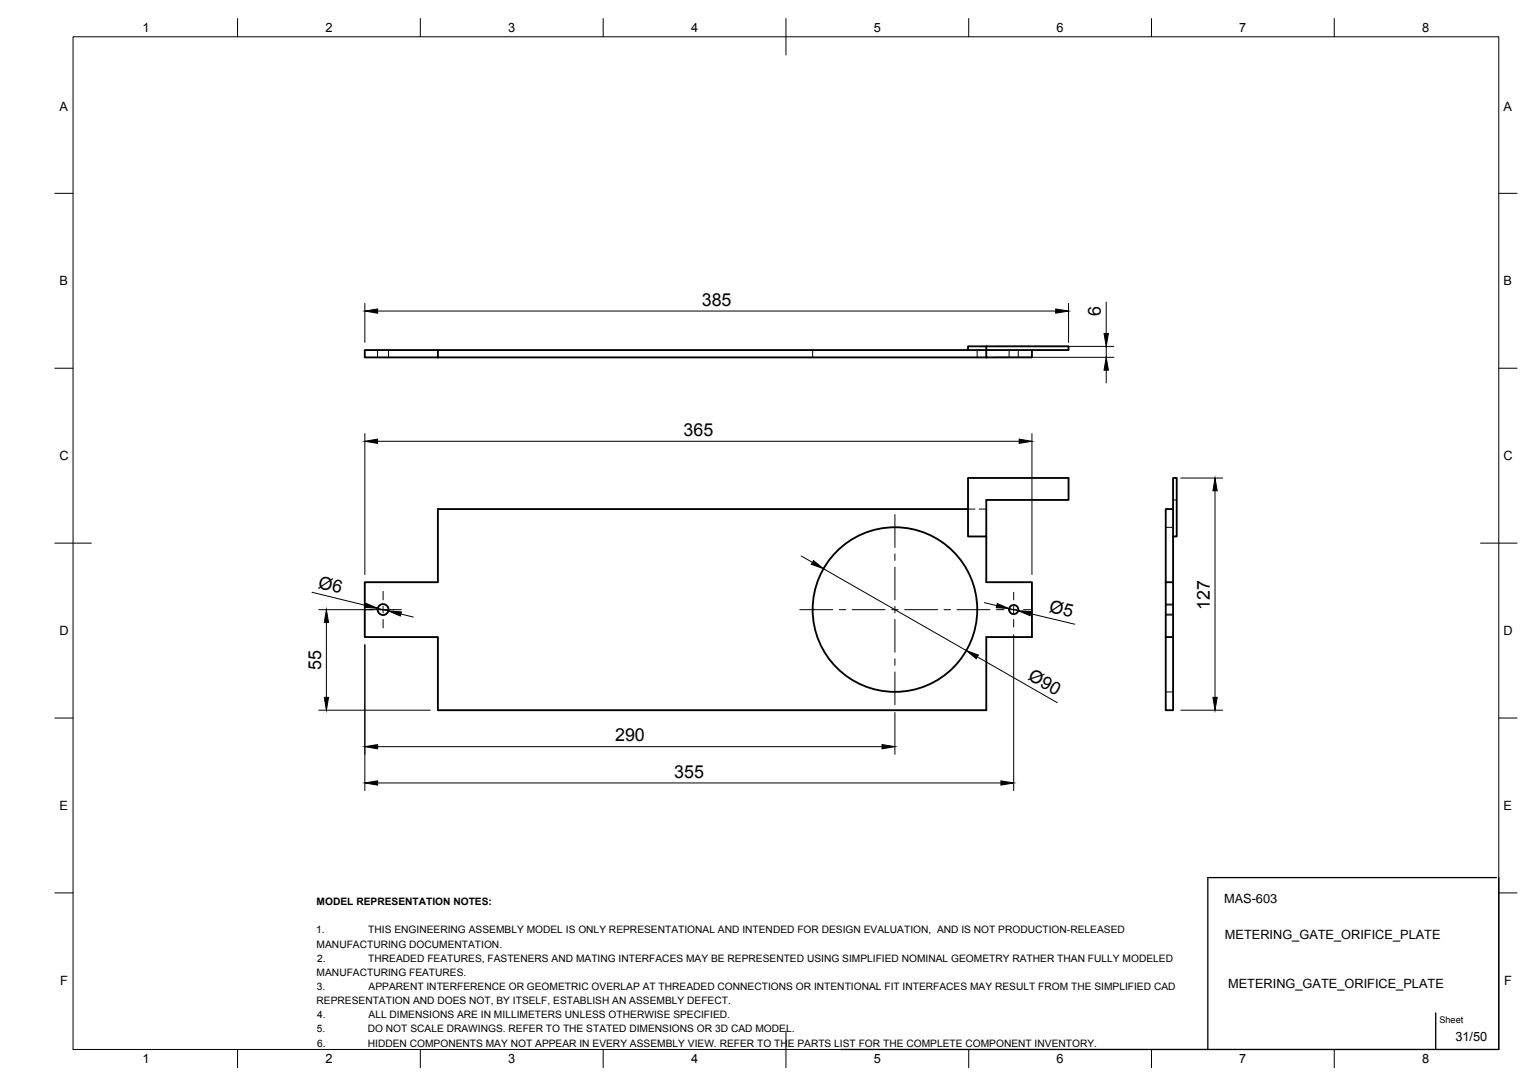
ISO-10303-21;
HEADER;
FILE_DESCRIPTION((''),'2;1');
FILE_NAME('METERING_GATE_ORIFICE_PLATE.step','2026-10-01T22:06:14-07:00',(''),(''),'','','');
FILE_SCHEMA (('AUTOMOTIVE_DESIGN { 1 0 10303 214 3 1 1 }'));
ENDSEC;
DATA;
#10=MECHANICAL_DESIGN_GEOMETRIC_PRESENTATION_REPRESENTATION('',(#1003),#50440);
#911=SHAPE_REPRESENTATION_RELATIONSHIP('SRR','None',#50644,#956) ;
#956=ADVANCED_BREP_SHAPE_REPRESENTATION('',(#1058),#50413) ;
#1003=STYLED_ITEM('',(#50889),#1058) ;
#1058=MANIFOLD_SOLID_BREP('METERING_GATE_ORIFICE_PLATE',#28670) ;
#1332=FACE_BOUND('',#5081,.T.) ;
#1333=FACE_BOUND('',#5082,.T.) ;
#1334=FACE_BOUND('',#5083,.T.) ;
#1335=FACE_BOUND('',#5085,.T.) ;
#1336=FACE_BOUND('',#5086,.T.) ;
#1337=FACE_BOUND('',#5087,.T.) ;
#2131=PLANE('',#30735) ;
#2132=PLANE('',#30736) ;
#2133=PLANE('',#30737) ;
#2134=PLANE('',#30738) ;
#2135=PLANE('',#30739) ;
#2136=PLANE('',#30740) ;
#2137=PLANE('',#30741) ;
#2138=PLANE('',#30745) ;
#2139=PLANE('',#30746) ;
#2140=PLANE('',#30747) ;
#2141=PLANE('',#30748) ;
#2142=PLANE('',#30749) ;
#2143=PLANE('',#30753) ;
#2144=PLANE('',#30754) ;
#2145=PLANE('',#30755) ;
#2146=PLANE('',#30756) ;
#2147=PLANE('',#30757) ;
#2148=PLANE('',#30761) ;
#2149=PLANE('',#30762) ;
#2150=PLANE('',#30763) ;
#2151=PLANE('',#30764) ;
#3286=FACE_OUTER_BOUND('',#5060,.T.) ;
#3287=FACE_OUTER_BOUND('',#5061,.T.) ;
#3288=FACE_OUTER_BOUND('',#5062,.T.) ;
#3289=FACE_OUTER_BOUND('',#5063,.T.) ;
#3290=FACE_OUTER_BOUND('',#5064,.T.) ;
#3291=FACE_OUTER_BOUND('',#5065,.T.) ;
#3292=FACE_OUTER_BOUND('',#5066,.T.) ;
#3293=FACE_OUTER_BOUND('',#5067,.T.) ;
#3294=FACE_OUTER_BOUND('',#5068,.T.) ;
#3295=FACE_OUTER_BOUND('',#5069,.T.) ;
#3296=FACE_OUTER_BOUND('',#5070,.T.) ;
#3297=FACE_OUTER_BOUND('',#5071,.T.) ;
#3298=FACE_OUTER_BOUND('',#5072,.T.) ;
#3299=FACE_OUTER_BOUND('',#5073,.T.) ;
#3300=FACE_OUTER_BOUND('',#5074,.T.) ;
#3301=FACE_OUTER_BOUND('',#5075,.T.) ;
#3302=FACE_OUTER_BOUND('',#5076,.T.) ;
#3303=FACE_OUTER_BOUND('',#5077,.T.) ;
#3304=FACE_OUTER_BOUND('',#5078,.T.) ;
#3305=FACE_OUTER_BOUND('',#5079,.T.) ;
#3306=FACE_OUTER_BOUND('',#5080,.T.) ;
#3307=FACE_OUTER_BOUND('',#5084,.T.) ;
#3308=FACE_OUTER_BOUND('',#5088,.T.) ;
#3309=FACE_OUTER_BOUND('',#5089,.T.) ;
#5060=EDGE_LOOP('',(#23447,#23448,#23449,#23450)) ;
#5061=EDGE_LOOP('',(#23451,#23452,#23453,#23454)) ;
#5062=EDGE_LOOP('',(#23455,#23456,#23457,#23458,#23459,#23460)) ;
#5063=EDGE_LOOP('',(#23461,#23462,#23463,#23464,#23465)) ;
#5064=EDGE_LOOP('',(#23466,#23467,#23468,#23469,#23470,#23471)) ;
#5065=EDGE_LOOP('',(#23472,#23473,#23474,#23475)) ;
#5066=EDGE_LOOP('',(#23476,#23477,#23478,#23479)) ;
#5067=EDGE_LOOP('',(#23480,#23481,#23482,#23483)) ;
#5068=EDGE_LOOP('',(#23484,#23485,#23486,#23487)) ;
#5069=EDGE_LOOP('',(#23488,#23489,#23490,#23491)) ;
#5070=EDGE_LOOP('',(#23492,#23493,#23494,#23495)) ;
#5071=EDGE_LOOP('',(#23496,#23497,#23498,#23499)) ;
#5072=EDGE_LOOP('',(#23500,#23501,#23502,#23503,#23504,#23505,#23506,#23507)) ;
#5073=EDGE_LOOP('',(#23508,#23509,#23510,#23511)) ;
#5074=EDGE_LOOP('',(#23512,#23513,#23514,#23515)) ;
#5075=EDGE_LOOP('',(#23516,#23517,#23518,#23519)) ;
#5076=EDGE_LOOP('',(#23520,#23521,#23522,#23523)) ;
#5077=EDGE_LOOP('',(#23524,#23525,#23526,#23527)) ;
#5078=EDGE_LOOP('',(#23528,#23529,#23530,#23531)) ;
#5079=EDGE_LOOP('',(#23532,#23533,#23534,#23535)) ;
#5080=EDGE_LOOP('',(#23536,#23537,#23538,#23539,#23540,#23541,#23542,#23543,
#23544,#23545,#23546,#23547,#23548,#23549)) ;
#5081=EDGE_LOOP('',(#23550)) ;
#5082=EDGE_LOOP('',(#23551)) ;
#5083=EDGE_LOOP('',(#23552)) ;
#5084=EDGE_LOOP('',(#23553,#23554,#23555,#23556,#23557,#23558,#23559,#23560,
#23561,#23562,#23563,#23564)) ;
#5085=EDGE_LOOP('',(#23565)) ;
#5086=EDGE_LOOP('',(#23566)) ;
#5087=EDGE_LOOP('',(#23567)) ;
#5088=EDGE_LOOP('',(#23568,#23569,#23570,#23571)) ;
#5089=EDGE_LOOP('',(#23572,#23573,#23574,#23575,#23576)) ;
#7620=LINE('',#46428,#10092) ;
#7621=LINE('',#46430,#10093) ;
#7622=LINE('',#46432,#10094) ;
#7623=LINE('',#46433,#10095) ;
#7624=LINE('',#46436,#10096) ;
#7625=LINE('',#46438,#10097) ;
#7626=LINE('',#46439,#10098) ;
#7627=LINE('',#46443,#10099) ;
#7628=LINE('',#46445,#10100) ;
#7629=LINE('',#46446,#10101) ;
#7630=LINE('',#46447,#10102) ;
#7631=LINE('',#46451,#10103) ;
#7632=LINE('',#46452,#10104) ;
#7633=LINE('',#46454,#10105) ;
#7634=LINE('',#46455,#10106) ;
#7635=LINE('',#46458,#10107) ;
#7636=LINE('',#46459,#10108) ;
#7637=LINE('',#46460,#10109) ;
#7638=LINE('',#46463,#10110) ;
#7639=LINE('',#46464,#10111) ;
#7640=LINE('',#46470,#10112) ;
#7641=LINE('',#46475,#10113) ;
#7642=LINE('',#46477,#10114) ;
#7643=LINE('',#46479,#10115) ;
#7644=LINE('',#46480,#10116) ;
#7645=LINE('',#46484,#10117) ;
#7646=LINE('',#46486,#10118) ;
#7647=LINE('',#46488,#10119) ;
#7648=LINE('',#46489,#10120) ;
#7649=LINE('',#46491,#10121) ;
#7650=LINE('',#46492,#10122) ;
#7651=LINE('',#46495,#10123) ;
#7652=LINE('',#46497,#10124) ;
#7653=LINE('',#46498,#10125) ;
#7654=LINE('',#46501,#10126) ;
#7655=LINE('',#46502,#10127) ;
#7656=LINE('',#46503,#10128) ;
#7657=LINE('',#46508,#10129) ;
#7658=LINE('',#46513,#10130) ;
#7659=LINE('',#46515,#10131) ;
#7660=LINE('',#46517,#10132) ;
#7661=LINE('',#46518,#10133) ;
#7662=LINE('',#46522,#10134) ;
#7663=LINE('',#46523,#10135) ;
#7664=LINE('',#46524,#10136) ;
#7665=LINE('',#46528,#10137) ;
#7666=LINE('',#46529,#10138) ;
#7667=LINE('',#46530,#10139) ;
#7668=LINE('',#46533,#10140) ;
#7669=LINE('',#46535,#10141) ;
#7670=LINE('',#46536,#10142) ;
#7671=LINE('',#46539,#10143) ;
#7672=LINE('',#46541,#10144) ;
#7673=LINE('',#46542,#10145) ;
#7674=LINE('',#46547,#10146) ;
#7675=LINE('',#46550,#10147) ;
#7676=LINE('',#46551,#10148) ;
#7677=LINE('',#46553,#10149) ;
#7678=LINE('',#46554,#10150) ;
#10092=VECTOR('',#37317,1.) ;
#10093=VECTOR('',#37318,1.) ;
#10094=VECTOR('',#37319,1.) ;
#10095=VECTOR('',#37320,1.) ;
#10096=VECTOR('',#37323,1.) ;
#10097=VECTOR('',#37324,1.) ;
#10098=VECTOR('',#37325,1.) ;
#10099=VECTOR('',#37328,1.) ;
#10100=VECTOR('',#37329,1.) ;
#10101=VECTOR('',#37330,1.) ;
#10102=VECTOR('',#37331,1.) ;
#10103=VECTOR('',#37334,1.) ;
#10104=VECTOR('',#37335,1.) ;
#10105=VECTOR('',#37336,1.) ;
#10106=VECTOR('',#37337,1.) ;
#10107=VECTOR('',#37340,1.) ;
#10108=VECTOR('',#37341,1.) ;
#10109=VECTOR('',#37342,1.) ;
#10110=VECTOR('',#37345,1.) ;
#10111=VECTOR('',#37346,1.) ;
#10112=VECTOR('',#37353,0.25) ;
#10113=VECTOR('',#37358,1.) ;
#10114=VECTOR('',#37359,1.) ;
#10115=VECTOR('',#37360,1.) ;
#10116=VECTOR('',#37361,1.) ;
#10117=VECTOR('',#37364,1.) ;
#10118=VECTOR('',#37365,1.) ;
#10119=VECTOR('',#37366,1.) ;
#10120=VECTOR('',#37367,1.) ;
#10121=VECTOR('',#37370,1.) ;
#10122=VECTOR('',#37371,1.) ;
#10123=VECTOR('',#37374,1.) ;
#10124=VECTOR('',#37375,1.) ;
#10125=VECTOR('',#37376,1.) ;
#10126=VECTOR('',#37379,1.) ;
#10127=VECTOR('',#37380,1.) ;
#10128=VECTOR('',#37381,1.) ;
#10129=VECTOR('',#37386,0.3) ;
#10130=VECTOR('',#37391,1.) ;
#10131=VECTOR('',#37392,1.) ;
#10132=VECTOR('',#37393,1.) ;
#10133=VECTOR('',#37394,1.) ;
#10134=VECTOR('',#37397,1.) ;
#10135=VECTOR('',#37398,1.) ;
#10136=VECTOR('',#37399,1.) ;
#10137=VECTOR('',#37402,1.) ;
#10138=VECTOR('',#37403,1.) ;
#10139=VECTOR('',#37404,1.) ;
#10140=VECTOR('',#37407,1.) ;
#10141=VECTOR('',#37408,1.) ;
#10142=VECTOR('',#37409,1.) ;
#10143=VECTOR('',#37412,1.) ;
#10144=VECTOR('',#37413,1.) ;
#10145=VECTOR('',#37414,1.) ;
#10146=VECTOR('',#37419,4.5) ;
#10147=VECTOR('',#37424,1.) ;
#10148=VECTOR('',#37425,1.) ;
#10149=VECTOR('',#37428,1.) ;
#10150=VECTOR('',#37429,1.) ;
#11173=CIRCLE('',#30743,0.25) ;
#11174=CIRCLE('',#30744,0.25) ;
#11175=CIRCLE('',#30751,0.3) ;
#11176=CIRCLE('',#30752,0.3) ;
#11177=CIRCLE('',#30759,4.5) ;
#11178=CIRCLE('',#30760,4.5) ;
#13465=VERTEX_POINT('',#46426) ;
#13466=VERTEX_POINT('',#46427) ;
#13467=VERTEX_POINT('',#46429) ;
#13468=VERTEX_POINT('',#46431) ;
#13469=VERTEX_POINT('',#46435) ;
#13470=VERTEX_POINT('',#46437) ;
#13471=VERTEX_POINT('',#46441) ;
#13472=VERTEX_POINT('',#46442) ;
#13473=VERTEX_POINT('',#46444) ;
#13474=VERTEX_POINT('',#46449) ;
#13475=VERTEX_POINT('',#46450) ;
#13476=VERTEX_POINT('',#46453) ;
#13477=VERTEX_POINT('',#46457) ;
#13478=VERTEX_POINT('',#46462) ;
#13479=VERTEX_POINT('',#46467) ;
#13480=VERTEX_POINT('',#46469) ;
#13481=VERTEX_POINT('',#46473) ;
#13482=VERTEX_POINT('',#46474) ;
#13483=VERTEX_POINT('',#46476) ;
#13484=VERTEX_POINT('',#46478) ;
#13485=VERTEX_POINT('',#46482) ;
#13486=VERTEX_POINT('',#46483) ;
#13487=VERTEX_POINT('',#46485) ;
#13488=VERTEX_POINT('',#46487) ;
#13489=VERTEX_POINT('',#46494) ;
#13490=VERTEX_POINT('',#46496) ;
#13491=VERTEX_POINT('',#46500) ;
#13492=VERTEX_POINT('',#46505) ;
#13493=VERTEX_POINT('',#46507) ;
#13494=VERTEX_POINT('',#46511) ;
#13495=VERTEX_POINT('',#46512) ;
#13496=VERTEX_POINT('',#46514) ;
#13497=VERTEX_POINT('',#46516) ;
#13498=VERTEX_POINT('',#46520) ;
#13499=VERTEX_POINT('',#46521) ;
#13500=VERTEX_POINT('',#46526) ;
#13501=VERTEX_POINT('',#46527) ;
#13502=VERTEX_POINT('',#46532) ;
#13503=VERTEX_POINT('',#46534) ;
#13504=VERTEX_POINT('',#46538) ;
#13505=VERTEX_POINT('',#46540) ;
#13506=VERTEX_POINT('',#46544) ;
#13507=VERTEX_POINT('',#46546) ;
#16989=EDGE_CURVE('',#13465,#13466,#7620,.T.) ;
#16990=EDGE_CURVE('',#13467,#13465,#7621,.T.) ;
#16991=EDGE_CURVE('',#13468,#13467,#7622,.T.) ;
#16992=EDGE_CURVE('',#13466,#13468,#7623,.T.) ;
#16993=EDGE_CURVE('',#13469,#13467,#7624,.T.) ;
#16994=EDGE_CURVE('',#13470,#13469,#7625,.T.) ;
#16995=EDGE_CURVE('',#13468,#13470,#7626,.T.) ;
#16996=EDGE_CURVE('',#13471,#13472,#7627,.T.) ;
#16997=EDGE_CURVE('',#13472,#13473,#7628,.T.) ;
#16998=EDGE_CURVE('',#13473,#13466,#7629,.T.) ;
#16999=EDGE_CURVE('',#13470,#13471,#7630,.T.) ;
#17000=EDGE_CURVE('',#13474,#13475,#7631,.T.) ;
#17001=EDGE_CURVE('',#13472,#13474,#7632,.T.) ;
#17002=EDGE_CURVE('',#13471,#13476,#7633,.T.) ;
#17003=EDGE_CURVE('',#13475,#13476,#7634,.T.) ;
#17004=EDGE_CURVE('',#13477,#13475,#7635,.T.) ;
#17005=EDGE_CURVE('',#13476,#13469,#7636,.T.) ;
#17006=EDGE_CURVE('',#13465,#13477,#7637,.T.) ;
#17007=EDGE_CURVE('',#13478,#13474,#7638,.T.) ;
#17008=EDGE_CURVE('',#13473,#13478,#7639,.T.) ;
#17009=EDGE_CURVE('',#13479,#13479,#11173,.T.) ;
#17010=EDGE_CURVE('',#13479,#13480,#7640,.T.) ;
#17011=EDGE_CURVE('',#13480,#13480,#11174,.T.) ;
#17012=EDGE_CURVE('',#13481,#13482,#7641,.T.) ;
#17013=EDGE_CURVE('',#13483,#13481,#7642,.T.) ;
#17014=EDGE_CURVE('',#13484,#13483,#7643,.T.) ;
#17015=EDGE_CURVE('',#13482,#13484,#7644,.T.) ;
#17016=EDGE_CURVE('',#13485,#13486,#7645,.T.) ;
#17017=EDGE_CURVE('',#13487,#13486,#7646,.T.) ;
#17018=EDGE_CURVE('',#13488,#13487,#7647,.T.) ;
#17019=EDGE_CURVE('',#13485,#13488,#7648,.T.) ;
#17020=EDGE_CURVE('',#13486,#13483,#7649,.T.) ;
#17021=EDGE_CURVE('',#13484,#13485,#7650,.T.) ;
#17022=EDGE_CURVE('',#13489,#13482,#7651,.T.) ;
#17023=EDGE_CURVE('',#13489,#13490,#7652,.T.) ;
#17024=EDGE_CURVE('',#13481,#13490,#7653,.T.) ;
#17025=EDGE_CURVE('',#13491,#13487,#7654,.T.) ;
#17026=EDGE_CURVE('',#13477,#13491,#7655,.T.) ;
#17027=EDGE_CURVE('',#13488,#13478,#7656,.T.) ;
#17028=EDGE_CURVE('',#13492,#13492,#11175,.T.) ;
#17029=EDGE_CURVE('',#13492,#13493,#7657,.T.) ;
#17030=EDGE_CURVE('',#13493,#13493,#11176,.T.) ;
#17031=EDGE_CURVE('',#13494,#13495,#7658,.T.) ;
#17032=EDGE_CURVE('',#13496,#13495,#7659,.T.) ;
#17033=EDGE_CURVE('',#13497,#13496,#7660,.T.) ;
#17034=EDGE_CURVE('',#13494,#13497,#7661,.T.) ;
#17035=EDGE_CURVE('',#13498,#13499,#7662,.T.) ;
#17036=EDGE_CURVE('',#13495,#13499,#7663,.T.) ;
#17037=EDGE_CURVE('',#13498,#13494,#7664,.T.) ;
#17038=EDGE_CURVE('',#13500,#13501,#7665,.T.) ;
#17039=EDGE_CURVE('',#13499,#13500,#7666,.T.) ;
#17040=EDGE_CURVE('',#13501,#13498,#7667,.T.) ;
#17041=EDGE_CURVE('',#13502,#13501,#7668,.T.) ;
#17042=EDGE_CURVE('',#13502,#13503,#7669,.T.) ;
#17043=EDGE_CURVE('',#13500,#13503,#7670,.T.) ;
#17044=EDGE_CURVE('',#13504,#13496,#7671,.T.) ;
#17045=EDGE_CURVE('',#13505,#13504,#7672,.T.) ;
#17046=EDGE_CURVE('',#13497,#13505,#7673,.T.) ;
#17047=EDGE_CURVE('',#13506,#13506,#11177,.T.) ;
#17048=EDGE_CURVE('',#13506,#13507,#7674,.T.) ;
#17049=EDGE_CURVE('',#13507,#13507,#11178,.T.) ;
#17050=EDGE_CURVE('',#13475,#13502,#7675,.T.) ;
#17051=EDGE_CURVE('',#13505,#13489,#7676,.T.) ;
#17052=EDGE_CURVE('',#13490,#13504,#7677,.T.) ;
#17053=EDGE_CURVE('',#13503,#13491,#7678,.T.) ;
#23447=ORIENTED_EDGE('',*,*,#16989,.F.) ;
#23448=ORIENTED_EDGE('',*,*,#16990,.F.) ;
#23449=ORIENTED_EDGE('',*,*,#16991,.F.) ;
#23450=ORIENTED_EDGE('',*,*,#16992,.F.) ;
#23451=ORIENTED_EDGE('',*,*,#16991,.T.) ;
#23452=ORIENTED_EDGE('',*,*,#16993,.F.) ;
#23453=ORIENTED_EDGE('',*,*,#16994,.F.) ;
#23454=ORIENTED_EDGE('',*,*,#16995,.F.) ;
#23455=ORIENTED_EDGE('',*,*,#16996,.T.) ;
#23456=ORIENTED_EDGE('',*,*,#16997,.T.) ;
#23457=ORIENTED_EDGE('',*,*,#16998,.T.) ;
#23458=ORIENTED_EDGE('',*,*,#16992,.T.) ;
#23459=ORIENTED_EDGE('',*,*,#16995,.T.) ;
#23460=ORIENTED_EDGE('',*,*,#16999,.T.) ;
#23461=ORIENTED_EDGE('',*,*,#17000,.F.) ;
#23462=ORIENTED_EDGE('',*,*,#17001,.F.) ;
#23463=ORIENTED_EDGE('',*,*,#16996,.F.) ;
#23464=ORIENTED_EDGE('',*,*,#17002,.T.) ;
#23465=ORIENTED_EDGE('',*,*,#17003,.F.) ;
#23466=ORIENTED_EDGE('',*,*,#17004,.T.) ;
#23467=ORIENTED_EDGE('',*,*,#17003,.T.) ;
#23468=ORIENTED_EDGE('',*,*,#17005,.T.) ;
#23469=ORIENTED_EDGE('',*,*,#16993,.T.) ;
#23470=ORIENTED_EDGE('',*,*,#16990,.T.) ;
#23471=ORIENTED_EDGE('',*,*,#17006,.T.) ;
#23472=ORIENTED_EDGE('',*,*,#17001,.T.) ;
#23473=ORIENTED_EDGE('',*,*,#17007,.F.) ;
#23474=ORIENTED_EDGE('',*,*,#17008,.F.) ;
#23475=ORIENTED_EDGE('',*,*,#16997,.F.) ;
#23476=ORIENTED_EDGE('',*,*,#17005,.F.) ;
#23477=ORIENTED_EDGE('',*,*,#17002,.F.) ;
#23478=ORIENTED_EDGE('',*,*,#16999,.F.) ;
#23479=ORIENTED_EDGE('',*,*,#16994,.T.) ;
#23480=ORIENTED_EDGE('',*,*,#17009,.F.) ;
#23481=ORIENTED_EDGE('',*,*,#17010,.T.) ;
#23482=ORIENTED_EDGE('',*,*,#17011,.F.) ;
#23483=ORIENTED_EDGE('',*,*,#17010,.F.) ;
#23484=ORIENTED_EDGE('',*,*,#17012,.F.) ;
#23485=ORIENTED_EDGE('',*,*,#17013,.F.) ;
#23486=ORIENTED_EDGE('',*,*,#17014,.F.) ;
#23487=ORIENTED_EDGE('',*,*,#17015,.F.) ;
#23488=ORIENTED_EDGE('',*,*,#17016,.T.) ;
#23489=ORIENTED_EDGE('',*,*,#17017,.F.) ;
#23490=ORIENTED_EDGE('',*,*,#17018,.F.) ;
#23491=ORIENTED_EDGE('',*,*,#17019,.F.) ;
#23492=ORIENTED_EDGE('',*,*,#17014,.T.) ;
#23493=ORIENTED_EDGE('',*,*,#17020,.F.) ;
#23494=ORIENTED_EDGE('',*,*,#17016,.F.) ;
#23495=ORIENTED_EDGE('',*,*,#17021,.F.) ;
#23496=ORIENTED_EDGE('',*,*,#17012,.T.) ;
#23497=ORIENTED_EDGE('',*,*,#17022,.F.) ;
#23498=ORIENTED_EDGE('',*,*,#17023,.T.) ;
#23499=ORIENTED_EDGE('',*,*,#17024,.F.) ;
#23500=ORIENTED_EDGE('',*,*,#17018,.T.) ;
#23501=ORIENTED_EDGE('',*,*,#17025,.F.) ;
#23502=ORIENTED_EDGE('',*,*,#17026,.F.) ;
#23503=ORIENTED_EDGE('',*,*,#17006,.F.) ;
#23504=ORIENTED_EDGE('',*,*,#16989,.T.) ;
#23505=ORIENTED_EDGE('',*,*,#16998,.F.) ;
#23506=ORIENTED_EDGE('',*,*,#17008,.T.) ;
#23507=ORIENTED_EDGE('',*,*,#17027,.F.) ;
#23508=ORIENTED_EDGE('',*,*,#17028,.F.) ;
#23509=ORIENTED_EDGE('',*,*,#17029,.T.) ;
#23510=ORIENTED_EDGE('',*,*,#17030,.F.) ;
#23511=ORIENTED_EDGE('',*,*,#17029,.F.) ;
#23512=ORIENTED_EDGE('',*,*,#17031,.T.) ;
#23513=ORIENTED_EDGE('',*,*,#17032,.F.) ;
#23514=ORIENTED_EDGE('',*,*,#17033,.F.) ;
#23515=ORIENTED_EDGE('',*,*,#17034,.F.) ;
#23516=ORIENTED_EDGE('',*,*,#17035,.T.) ;
#23517=ORIENTED_EDGE('',*,*,#17036,.F.) ;
#23518=ORIENTED_EDGE('',*,*,#17031,.F.) ;
#23519=ORIENTED_EDGE('',*,*,#17037,.F.) ;
#23520=ORIENTED_EDGE('',*,*,#17038,.F.) ;
#23521=ORIENTED_EDGE('',*,*,#17039,.F.) ;
#23522=ORIENTED_EDGE('',*,*,#17035,.F.) ;
#23523=ORIENTED_EDGE('',*,*,#17040,.F.) ;
#23524=ORIENTED_EDGE('',*,*,#17038,.T.) ;
#23525=ORIENTED_EDGE('',*,*,#17041,.F.) ;
#23526=ORIENTED_EDGE('',*,*,#17042,.T.) ;
#23527=ORIENTED_EDGE('',*,*,#17043,.F.) ;
#23528=ORIENTED_EDGE('',*,*,#17033,.T.) ;
#23529=ORIENTED_EDGE('',*,*,#17044,.F.) ;
#23530=ORIENTED_EDGE('',*,*,#17045,.F.) ;
#23531=ORIENTED_EDGE('',*,*,#17046,.F.) ;
#23532=ORIENTED_EDGE('',*,*,#17047,.F.) ;
#23533=ORIENTED_EDGE('',*,*,#17048,.T.) ;
#23534=ORIENTED_EDGE('',*,*,#17049,.F.) ;
#23535=ORIENTED_EDGE('',*,*,#17048,.F.) ;
#23536=ORIENTED_EDGE('',*,*,#17000,.T.) ;
#23537=ORIENTED_EDGE('',*,*,#17050,.T.) ;
#23538=ORIENTED_EDGE('',*,*,#17041,.T.) ;
#23539=ORIENTED_EDGE('',*,*,#17040,.T.) ;
#23540=ORIENTED_EDGE('',*,*,#17037,.T.) ;
#23541=ORIENTED_EDGE('',*,*,#17034,.T.) ;
#23542=ORIENTED_EDGE('',*,*,#17046,.T.) ;
#23543=ORIENTED_EDGE('',*,*,#17051,.T.) ;
#23544=ORIENTED_EDGE('',*,*,#17022,.T.) ;
#23545=ORIENTED_EDGE('',*,*,#17015,.T.) ;
#23546=ORIENTED_EDGE('',*,*,#17021,.T.) ;
#23547=ORIENTED_EDGE('',*,*,#17019,.T.) ;
#23548=ORIENTED_EDGE('',*,*,#17027,.T.) ;
#23549=ORIENTED_EDGE('',*,*,#17007,.T.) ;
#23550=ORIENTED_EDGE('',*,*,#17011,.T.) ;
#23551=ORIENTED_EDGE('',*,*,#17030,.T.) ;
#23552=ORIENTED_EDGE('',*,*,#17049,.T.) ;
#23553=ORIENTED_EDGE('',*,*,#17025,.T.) ;
#23554=ORIENTED_EDGE('',*,*,#17017,.T.) ;
#23555=ORIENTED_EDGE('',*,*,#17020,.T.) ;
#23556=ORIENTED_EDGE('',*,*,#17013,.T.) ;
#23557=ORIENTED_EDGE('',*,*,#17024,.T.) ;
#23558=ORIENTED_EDGE('',*,*,#17052,.T.) ;
#23559=ORIENTED_EDGE('',*,*,#17044,.T.) ;
#23560=ORIENTED_EDGE('',*,*,#17032,.T.) ;
#23561=ORIENTED_EDGE('',*,*,#17036,.T.) ;
#23562=ORIENTED_EDGE('',*,*,#17039,.T.) ;
#23563=ORIENTED_EDGE('',*,*,#17043,.T.) ;
#23564=ORIENTED_EDGE('',*,*,#17053,.T.) ;
#23565=ORIENTED_EDGE('',*,*,#17009,.T.) ;
#23566=ORIENTED_EDGE('',*,*,#17028,.T.) ;
#23567=ORIENTED_EDGE('',*,*,#17047,.T.) ;
#23568=ORIENTED_EDGE('',*,*,#17045,.T.) ;
#23569=ORIENTED_EDGE('',*,*,#17052,.F.) ;
#23570=ORIENTED_EDGE('',*,*,#17023,.F.) ;
#23571=ORIENTED_EDGE('',*,*,#17051,.F.) ;
#23572=ORIENTED_EDGE('',*,*,#17026,.T.) ;
#23573=ORIENTED_EDGE('',*,*,#17053,.F.) ;
#23574=ORIENTED_EDGE('',*,*,#17042,.F.) ;
#23575=ORIENTED_EDGE('',*,*,#17050,.F.) ;
#23576=ORIENTED_EDGE('',*,*,#17004,.F.) ;
#26844=CYLINDRICAL_SURFACE('',#30742,0.25) ;
#26845=CYLINDRICAL_SURFACE('',#30750,0.3) ;
#26846=CYLINDRICAL_SURFACE('',#30758,4.5) ;
#28021=ADVANCED_FACE('',(#3286),#2131,.F.) ;
#28022=ADVANCED_FACE('',(#3287),#2132,.F.) ;
#28023=ADVANCED_FACE('',(#3288),#2133,.T.) ;
#28024=ADVANCED_FACE('',(#3289),#2134,.F.) ;
#28025=ADVANCED_FACE('',(#3290),#2135,.F.) ;
#28026=ADVANCED_FACE('',(#3291),#2136,.F.) ;
#28027=ADVANCED_FACE('',(#3292),#2137,.F.) ;
#28028=ADVANCED_FACE('',(#3293),#26844,.F.) ;
#28029=ADVANCED_FACE('',(#3294),#2138,.F.) ;
#28030=ADVANCED_FACE('',(#3295),#2139,.F.) ;
#28031=ADVANCED_FACE('',(#3296),#2140,.F.) ;
#28032=ADVANCED_FACE('',(#3297),#2141,.F.) ;
#28033=ADVANCED_FACE('',(#3298),#2142,.F.) ;
#28034=ADVANCED_FACE('',(#3299),#26845,.F.) ;
#28035=ADVANCED_FACE('',(#3300),#2143,.F.) ;
#28036=ADVANCED_FACE('',(#3301),#2144,.F.) ;
#28037=ADVANCED_FACE('',(#3302),#2145,.F.) ;
#28038=ADVANCED_FACE('',(#3303),#2146,.F.) ;
#28039=ADVANCED_FACE('',(#3304),#2147,.F.) ;
#28040=ADVANCED_FACE('',(#3305),#26846,.F.) ;
#28041=ADVANCED_FACE('',(#3306,#1332,#1333,#1334),#2148,.T.) ;
#28042=ADVANCED_FACE('',(#3307,#1335,#1336,#1337),#2149,.F.) ;
#28043=ADVANCED_FACE('',(#3308),#2150,.F.) ;
#28044=ADVANCED_FACE('',(#3309),#2151,.F.) ;
#28670=CLOSED_SHELL('',(#28021,#28022,#28023,#28024,#28025,#28026,#28027,
#28028,#28029,#28030,#28031,#28032,#28033,#28034,#28035,#28036,#28037,#28038,
#28039,#28040,#28041,#28042,#28043,#28044)) ;
#30734=AXIS2_PLACEMENT_3D('',#46424,#37313,#37314) ;
#30735=AXIS2_PLACEMENT_3D('',#46425,#37315,#37316) ;
#30736=AXIS2_PLACEMENT_3D('',#46434,#37321,#37322) ;
#30737=AXIS2_PLACEMENT_3D('',#46440,#37326,#37327) ;
#30738=AXIS2_PLACEMENT_3D('',#46448,#37332,#37333) ;
#30739=AXIS2_PLACEMENT_3D('',#46456,#37338,#37339) ;
#30740=AXIS2_PLACEMENT_3D('',#46461,#37343,#37344) ;
#30741=AXIS2_PLACEMENT_3D('',#46465,#37347,#37348) ;
#30742=AXIS2_PLACEMENT_3D('',#46466,#37349,#37350) ;
#30743=AXIS2_PLACEMENT_3D('',#46468,#37351,#37352) ;
#30744=AXIS2_PLACEMENT_3D('',#46471,#37354,#37355) ;
#30745=AXIS2_PLACEMENT_3D('',#46472,#37356,#37357) ;
#30746=AXIS2_PLACEMENT_3D('',#46481,#37362,#37363) ;
#30747=AXIS2_PLACEMENT_3D('',#46490,#37368,#37369) ;
#30748=AXIS2_PLACEMENT_3D('',#46493,#37372,#37373) ;
#30749=AXIS2_PLACEMENT_3D('',#46499,#37377,#37378) ;
#30750=AXIS2_PLACEMENT_3D('',#46504,#37382,#37383) ;
#30751=AXIS2_PLACEMENT_3D('',#46506,#37384,#37385) ;
#30752=AXIS2_PLACEMENT_3D('',#46509,#37387,#37388) ;
#30753=AXIS2_PLACEMENT_3D('',#46510,#37389,#37390) ;
#30754=AXIS2_PLACEMENT_3D('',#46519,#37395,#37396) ;
#30755=AXIS2_PLACEMENT_3D('',#46525,#37400,#37401) ;
#30756=AXIS2_PLACEMENT_3D('',#46531,#37405,#37406) ;
#30757=AXIS2_PLACEMENT_3D('',#46537,#37410,#37411) ;
#30758=AXIS2_PLACEMENT_3D('',#46543,#37415,#37416) ;
#30759=AXIS2_PLACEMENT_3D('',#46545,#37417,#37418) ;
#30760=AXIS2_PLACEMENT_3D('',#46548,#37420,#37421) ;
#30761=AXIS2_PLACEMENT_3D('',#46549,#37422,#37423) ;
#30762=AXIS2_PLACEMENT_3D('',#46552,#37426,#37427) ;
#30763=AXIS2_PLACEMENT_3D('',#46555,#37430,#37431) ;
#30764=AXIS2_PLACEMENT_3D('',#46556,#37432,#37433) ;
#37313=DIRECTION('axis',(0.,0.,1.)) ;
#37314=DIRECTION('refdir',(1.,0.,0.)) ;
#37315=DIRECTION('center_axis',(0.,1.,0.)) ;
#37316=DIRECTION('ref_axis',(0.,0.,1.)) ;
#37317=DIRECTION('',(0.,0.,1.)) ;
#37318=DIRECTION('',(-1.,0.,0.)) ;
#37319=DIRECTION('',(0.,0.,-1.)) ;
#37320=DIRECTION('',(1.,0.,0.)) ;
#37321=DIRECTION('center_axis',(-1.,0.,0.)) ;
#37322=DIRECTION('ref_axis',(0.,0.,1.)) ;
#37323=DIRECTION('',(0.,-1.,0.)) ;
#37324=DIRECTION('',(0.,0.,-1.)) ;
#37325=DIRECTION('',(0.,1.,0.)) ;
#37326=DIRECTION('center_axis',(0.,0.,1.)) ;
#37327=DIRECTION('ref_axis',(1.,0.,0.)) ;
#37328=DIRECTION('',(0.,-1.,0.)) ;
#37329=DIRECTION('',(1.,0.,0.)) ;
#37330=DIRECTION('',(0.,1.,0.)) ;
#37331=DIRECTION('',(-1.,0.,0.)) ;
#37332=DIRECTION('center_axis',(1.,0.,0.)) ;
#37333=DIRECTION('ref_axis',(0.,0.,-1.)) ;
#37334=DIRECTION('',(0.,1.,0.)) ;
#37335=DIRECTION('',(0.,0.,-1.)) ;
#37336=DIRECTION('',(0.,0.,-1.)) ;
#37337=DIRECTION('',(0.,1.,0.)) ;
#37338=DIRECTION('center_axis',(0.,0.,1.)) ;
#37339=DIRECTION('ref_axis',(1.,0.,0.)) ;
#37340=DIRECTION('',(-1.,0.,0.)) ;
#37341=DIRECTION('',(1.,0.,0.)) ;
#37342=DIRECTION('',(0.,-1.,0.)) ;
#37343=DIRECTION('center_axis',(0.,1.,0.)) ;
#37344=DIRECTION('ref_axis',(0.,0.,1.)) ;
#37345=DIRECTION('',(-1.,0.,0.)) ;
#37346=DIRECTION('',(0.,0.,-1.)) ;
#37347=DIRECTION('center_axis',(0.,-1.,0.)) ;
#37348=DIRECTION('ref_axis',(0.,0.,-1.)) ;
#37349=DIRECTION('center_axis',(0.,0.,1.)) ;
#37350=DIRECTION('ref_axis',(1.,0.,0.)) ;
#37351=DIRECTION('center_axis',(0.,0.,1.)) ;
#37352=DIRECTION('ref_axis',(1.,0.,0.)) ;
#37353=DIRECTION('',(0.,0.,1.)) ;
#37354=DIRECTION('center_axis',(0.,0.,-1.)) ;
#37355=DIRECTION('ref_axis',(1.,0.,0.)) ;
#37356=DIRECTION('center_axis',(0.,1.,0.)) ;
#37357=DIRECTION('ref_axis',(0.,0.,1.)) ;
#37358=DIRECTION('',(0.,0.,1.)) ;
#37359=DIRECTION('',(-1.,0.,0.)) ;
#37360=DIRECTION('',(0.,0.,-1.)) ;
#37361=DIRECTION('',(1.,0.,0.)) ;
#37362=DIRECTION('center_axis',(0.,-1.,0.)) ;
#37363=DIRECTION('ref_axis',(0.,0.,-1.)) ;
#37364=DIRECTION('',(0.,0.,-1.)) ;
#37365=DIRECTION('',(1.,0.,0.)) ;
#37366=DIRECTION('',(0.,0.,-1.)) ;
#37367=DIRECTION('',(-1.,0.,0.)) ;
#37368=DIRECTION('center_axis',(-1.,0.,0.)) ;
#37369=DIRECTION('ref_axis',(0.,0.,1.)) ;
#37370=DIRECTION('',(0.,-1.,0.)) ;
#37371=DIRECTION('',(0.,1.,0.)) ;
#37372=DIRECTION('center_axis',(-1.,0.,0.)) ;
#37373=DIRECTION('ref_axis',(0.,0.,1.)) ;
#37374=DIRECTION('',(0.,1.,0.)) ;
#37375=DIRECTION('',(0.,0.,-1.)) ;
#37376=DIRECTION('',(0.,-1.,0.)) ;
#37377=DIRECTION('center_axis',(-1.,0.,0.)) ;
#37378=DIRECTION('ref_axis',(0.,0.,1.)) ;
#37379=DIRECTION('',(0.,-1.,0.)) ;
#37380=DIRECTION('',(0.,0.,-1.)) ;
#37381=DIRECTION('',(0.,1.,0.)) ;
#37382=DIRECTION('center_axis',(0.,0.,1.)) ;
#37383=DIRECTION('ref_axis',(1.,0.,0.)) ;
#37384=DIRECTION('center_axis',(0.,0.,1.)) ;
#37385=DIRECTION('ref_axis',(1.,0.,0.)) ;
#37386=DIRECTION('',(0.,0.,1.)) ;
#37387=DIRECTION('center_axis',(0.,0.,-1.)) ;
#37388=DIRECTION('ref_axis',(1.,0.,0.)) ;
#37389=DIRECTION('center_axis',(0.,1.,0.)) ;
#37390=DIRECTION('ref_axis',(0.,0.,1.)) ;
#37391=DIRECTION('',(0.,0.,-1.)) ;
#37392=DIRECTION('',(-1.,0.,0.)) ;
#37393=DIRECTION('',(0.,0.,-1.)) ;
#37394=DIRECTION('',(1.,0.,0.)) ;
#37395=DIRECTION('center_axis',(1.,0.,0.)) ;
#37396=DIRECTION('ref_axis',(0.,0.,-1.)) ;
#37397=DIRECTION('',(0.,0.,-1.)) ;
#37398=DIRECTION('',(0.,1.,0.)) ;
#37399=DIRECTION('',(0.,-1.,0.)) ;
#37400=DIRECTION('center_axis',(0.,-1.,0.)) ;
#37401=DIRECTION('ref_axis',(0.,0.,-1.)) ;
#37402=DIRECTION('',(0.,0.,1.)) ;
#37403=DIRECTION('',(1.,0.,0.)) ;
#37404=DIRECTION('',(-1.,0.,0.)) ;
#37405=DIRECTION('center_axis',(1.,0.,0.)) ;
#37406=DIRECTION('ref_axis',(0.,0.,-1.)) ;
#37407=DIRECTION('',(0.,-1.,0.)) ;
#37408=DIRECTION('',(0.,0.,-1.)) ;
#37409=DIRECTION('',(0.,1.,0.)) ;
#37410=DIRECTION('center_axis',(1.,0.,0.)) ;
#37411=DIRECTION('ref_axis',(0.,0.,-1.)) ;
#37412=DIRECTION('',(0.,1.,0.)) ;
#37413=DIRECTION('',(0.,0.,-1.)) ;
#37414=DIRECTION('',(0.,-1.,0.)) ;
#37415=DIRECTION('center_axis',(0.,0.,1.)) ;
#37416=DIRECTION('ref_axis',(1.,0.,0.)) ;
#37417=DIRECTION('center_axis',(0.,0.,1.)) ;
#37418=DIRECTION('ref_axis',(1.,0.,0.)) ;
#37419=DIRECTION('',(0.,0.,1.)) ;
#37420=DIRECTION('center_axis',(0.,0.,-1.)) ;
#37421=DIRECTION('ref_axis',(1.,0.,0.)) ;
#37422=DIRECTION('center_axis',(0.,0.,1.)) ;
#37423=DIRECTION('ref_axis',(1.,0.,0.)) ;
#37424=DIRECTION('',(-1.,0.,0.)) ;
#37425=DIRECTION('',(1.,0.,0.)) ;
#37426=DIRECTION('center_axis',(0.,0.,1.)) ;
#37427=DIRECTION('ref_axis',(1.,0.,0.)) ;
#37428=DIRECTION('',(-1.,0.,0.)) ;
#37429=DIRECTION('',(1.,0.,0.)) ;
#37430=DIRECTION('center_axis',(0.,1.,0.)) ;
#37431=DIRECTION('ref_axis',(0.,0.,1.)) ;
#37432=DIRECTION('center_axis',(0.,-1.,0.)) ;
#37433=DIRECTION('ref_axis',(0.,0.,-1.)) ;
#46424=CARTESIAN_POINT('',(0.,0.,0.)) ;
#46425=CARTESIAN_POINT('Origin',(21.75,6.,42.9)) ;
#46426=CARTESIAN_POINT('',(20.,6.,42.8)) ;
#46427=CARTESIAN_POINT('',(20.,6.,43.)) ;
#46428=CARTESIAN_POINT('',(20.,6.,42.9)) ;
#46429=CARTESIAN_POINT('',(24.5,6.,42.8)) ;
#46430=CARTESIAN_POINT('',(21.75,6.,42.8)) ;
#46431=CARTESIAN_POINT('',(24.5,6.,43.)) ;
#46432=CARTESIAN_POINT('',(24.5,6.,42.9)) ;
#46433=CARTESIAN_POINT('',(21.75,6.,43.)) ;
#46434=CARTESIAN_POINT('Origin',(24.5,6.6,42.9)) ;
#46435=CARTESIAN_POINT('',(24.5,7.2,42.8)) ;
#46436=CARTESIAN_POINT('',(24.5,6.6,42.8)) ;
#46437=CARTESIAN_POINT('',(24.5,7.2,43.)) ;
#46438=CARTESIAN_POINT('',(24.5,7.2,42.9)) ;
#46439=CARTESIAN_POINT('',(24.5,6.6,43.)) ;
#46440=CARTESIAN_POINT('Origin',(19.5,5.6,43.)) ;
#46441=CARTESIAN_POINT('',(19.,7.2,43.)) ;
#46442=CARTESIAN_POINT('',(19.,4.,43.)) ;
#46443=CARTESIAN_POINT('',(19.,5.6,43.)) ;
#46444=CARTESIAN_POINT('',(20.,4.,43.)) ;
#46445=CARTESIAN_POINT('',(19.5,4.,43.)) ;
#46446=CARTESIAN_POINT('',(20.,5.6,43.)) ;
#46447=CARTESIAN_POINT('',(19.5,7.2,43.)) ;
#46448=CARTESIAN_POINT('Origin',(19.,5.6,42.9)) ;
#46449=CARTESIAN_POINT('',(19.,4.,42.8)) ;
#46450=CARTESIAN_POINT('',(19.,5.5,42.8)) ;
#46451=CARTESIAN_POINT('',(19.,2.8,42.8)) ;
#46452=CARTESIAN_POINT('',(19.,4.,42.9)) ;
#46453=CARTESIAN_POINT('',(19.,7.2,42.8)) ;
#46454=CARTESIAN_POINT('',(19.,7.2,42.9)) ;
#46455=CARTESIAN_POINT('',(19.,5.6,42.8)) ;
#46456=CARTESIAN_POINT('Origin',(19.5,5.6,42.8)) ;
#46457=CARTESIAN_POINT('',(20.,5.5,42.8)) ;
#46458=CARTESIAN_POINT('',(5.,5.5,42.8)) ;
#46459=CARTESIAN_POINT('',(21.75,7.2,42.8)) ;
#46460=CARTESIAN_POINT('',(20.,5.6,42.8)) ;
#46461=CARTESIAN_POINT('Origin',(19.5,4.,42.9)) ;
#46462=CARTESIAN_POINT('',(20.,4.,42.8)) ;
#46463=CARTESIAN_POINT('',(12.25,4.,42.8)) ;
#46464=CARTESIAN_POINT('',(20.,4.,42.9)) ;
#46465=CARTESIAN_POINT('Origin',(19.5,7.2,42.9)) ;
#46466=CARTESIAN_POINT('Origin',(21.5,0.,42.6)) ;
#46467=CARTESIAN_POINT('',(21.25,-3.06161699786838E-17,42.4)) ;
#46468=CARTESIAN_POINT('Origin',(21.5,0.,42.4)) ;
#46469=CARTESIAN_POINT('',(21.25,3.06161699786838E-17,42.8)) ;
#46470=CARTESIAN_POINT('',(21.25,-3.06161699786838E-17,42.6)) ;
#46471=CARTESIAN_POINT('Origin',(21.5,0.,42.8)) ;
#46472=CARTESIAN_POINT('Origin',(21.25,-1.5,42.6)) ;
#46473=CARTESIAN_POINT('',(20.,-1.5,42.4)) ;
#46474=CARTESIAN_POINT('',(20.,-1.5,42.8)) ;
#46475=CARTESIAN_POINT('',(20.,-1.5,42.6)) ;
#46476=CARTESIAN_POINT('',(22.5,-1.5,42.4)) ;
#46477=CARTESIAN_POINT('',(21.25,-1.5,42.4)) ;
#46478=CARTESIAN_POINT('',(22.5,-1.5,42.8)) ;
#46479=CARTESIAN_POINT('',(22.5,-1.5,42.6)) ;
#46480=CARTESIAN_POINT('',(21.25,-1.5,42.8)) ;
#46481=CARTESIAN_POINT('Origin',(21.25,1.5,42.6)) ;
#46482=CARTESIAN_POINT('',(22.5,1.5,42.8)) ;
#46483=CARTESIAN_POINT('',(22.5,1.5,42.4)) ;
#46484=CARTESIAN_POINT('',(22.5,1.5,42.6)) ;
#46485=CARTESIAN_POINT('',(20.,1.5,42.4)) ;
#46486=CARTESIAN_POINT('',(21.25,1.5,42.4)) ;
#46487=CARTESIAN_POINT('',(20.,1.5,42.8)) ;
#46488=CARTESIAN_POINT('',(20.,1.5,42.6)) ;
#46489=CARTESIAN_POINT('',(21.25,1.5,42.8)) ;
#46490=CARTESIAN_POINT('Origin',(22.5,0.,42.6)) ;
#46491=CARTESIAN_POINT('',(22.5,0.,42.4)) ;
#46492=CARTESIAN_POINT('',(22.5,0.,42.8)) ;
#46493=CARTESIAN_POINT('Origin',(20.,0.,42.6)) ;
#46494=CARTESIAN_POINT('',(20.,-5.5,42.8)) ;
#46495=CARTESIAN_POINT('',(20.,0.,42.8)) ;
#46496=CARTESIAN_POINT('',(20.,-5.5,42.4)) ;
#46497=CARTESIAN_POINT('',(20.,-5.5,42.6)) ;
#46498=CARTESIAN_POINT('',(20.,0.,42.4)) ;
#46499=CARTESIAN_POINT('Origin',(20.,0.,42.6)) ;
#46500=CARTESIAN_POINT('',(20.,5.5,42.4)) ;
#46501=CARTESIAN_POINT('',(20.,0.,42.4)) ;
#46502=CARTESIAN_POINT('',(20.,5.5,42.6)) ;
#46503=CARTESIAN_POINT('',(20.,0.,42.8)) ;
#46504=CARTESIAN_POINT('Origin',(-13.,0.,42.6)) ;
#46505=CARTESIAN_POINT('',(-13.3,-3.67394039744206E-17,42.4)) ;
#46506=CARTESIAN_POINT('Origin',(-13.,0.,42.4)) ;
#46507=CARTESIAN_POINT('',(-13.3,3.67394039744206E-17,42.8)) ;
#46508=CARTESIAN_POINT('',(-13.3,-3.67394039744206E-17,42.6)) ;
#46509=CARTESIAN_POINT('Origin',(-13.,0.,42.8)) ;
#46510=CARTESIAN_POINT('Origin',(-12.,-1.5,42.6)) ;
#46511=CARTESIAN_POINT('',(-14.,-1.5,42.8)) ;
#46512=CARTESIAN_POINT('',(-14.,-1.5,42.4)) ;
#46513=CARTESIAN_POINT('',(-14.,-1.5,42.6)) ;
#46514=CARTESIAN_POINT('',(-10.,-1.5,42.4)) ;
#46515=CARTESIAN_POINT('',(-12.,-1.5,42.4)) ;
#46516=CARTESIAN_POINT('',(-10.,-1.5,42.8)) ;
#46517=CARTESIAN_POINT('',(-10.,-1.5,42.6)) ;
#46518=CARTESIAN_POINT('',(-12.,-1.5,42.8)) ;
#46519=CARTESIAN_POINT('Origin',(-14.,0.,42.6)) ;
#46520=CARTESIAN_POINT('',(-14.,1.5,42.8)) ;
#46521=CARTESIAN_POINT('',(-14.,1.5,42.4)) ;
#46522=CARTESIAN_POINT('',(-14.,1.5,42.6)) ;
#46523=CARTESIAN_POINT('',(-14.,0.,42.4)) ;
#46524=CARTESIAN_POINT('',(-14.,0.,42.8)) ;
#46525=CARTESIAN_POINT('Origin',(-12.,1.5,42.6)) ;
#46526=CARTESIAN_POINT('',(-10.,1.5,42.4)) ;
#46527=CARTESIAN_POINT('',(-10.,1.5,42.8)) ;
#46528=CARTESIAN_POINT('',(-10.,1.5,42.6)) ;
#46529=CARTESIAN_POINT('',(-12.,1.5,42.4)) ;
#46530=CARTESIAN_POINT('',(-12.,1.5,42.8)) ;
#46531=CARTESIAN_POINT('Origin',(-10.,0.,42.6)) ;
#46532=CARTESIAN_POINT('',(-10.,5.5,42.8)) ;
#46533=CARTESIAN_POINT('',(-10.,0.,42.8)) ;
#46534=CARTESIAN_POINT('',(-10.,5.5,42.4)) ;
#46535=CARTESIAN_POINT('',(-10.,5.5,42.6)) ;
#46536=CARTESIAN_POINT('',(-10.,0.,42.4)) ;
#46537=CARTESIAN_POINT('Origin',(-10.,0.,42.6)) ;
#46538=CARTESIAN_POINT('',(-10.,-5.5,42.4)) ;
#46539=CARTESIAN_POINT('',(-10.,0.,42.4)) ;
#46540=CARTESIAN_POINT('',(-10.,-5.5,42.8)) ;
#46541=CARTESIAN_POINT('',(-10.,-5.5,42.6)) ;
#46542=CARTESIAN_POINT('',(-10.,0.,42.8)) ;
#46543=CARTESIAN_POINT('Origin',(15.,0.,42.6)) ;
#46544=CARTESIAN_POINT('',(10.5,-5.51091059616309E-16,42.4)) ;
#46545=CARTESIAN_POINT('Origin',(15.,0.,42.4)) ;
#46546=CARTESIAN_POINT('',(10.5,5.51091059616309E-16,42.8)) ;
#46547=CARTESIAN_POINT('',(10.5,-5.51091059616309E-16,42.6)) ;
#46548=CARTESIAN_POINT('Origin',(15.,0.,42.8)) ;
#46549=CARTESIAN_POINT('Origin',(5.,0.,42.8)) ;
#46550=CARTESIAN_POINT('',(5.,5.5,42.8)) ;
#46551=CARTESIAN_POINT('',(5.,-5.5,42.8)) ;
#46552=CARTESIAN_POINT('Origin',(5.,0.,42.4)) ;
#46553=CARTESIAN_POINT('',(5.,-5.5,42.4)) ;
#46554=CARTESIAN_POINT('',(5.,5.5,42.4)) ;
#46555=CARTESIAN_POINT('Origin',(5.,-5.5,42.6)) ;
#46556=CARTESIAN_POINT('Origin',(5.,5.5,42.6)) ;
#50360=UNCERTAINTY_MEASURE_WITH_UNIT(LENGTH_MEASURE(0.001),#50441,
'DISTANCE_ACCURACY_VALUE',
'Maximum model space distance between geometric entities at asserted c
onnectivities') ;
#50387=UNCERTAINTY_MEASURE_WITH_UNIT(LENGTH_MEASURE(0.001),#50441,
'DISTANCE_ACCURACY_VALUE',
'Maximum model space distance between geometric entities at asserted c
onnectivities') ;
#50413=(
GEOMETRIC_REPRESENTATION_CONTEXT(3)
GLOBAL_UNCERTAINTY_ASSIGNED_CONTEXT((#50360))
GLOBAL_UNIT_ASSIGNED_CONTEXT((#50441,#50443,#50444))
REPRESENTATION_CONTEXT('','3D')
) ;
#50440=(
GEOMETRIC_REPRESENTATION_CONTEXT(3)
GLOBAL_UNCERTAINTY_ASSIGNED_CONTEXT((#50387))
GLOBAL_UNIT_ASSIGNED_CONTEXT((#50441,#50443,#50444))
REPRESENTATION_CONTEXT('','3D')
) ;
#50441=(
LENGTH_UNIT()
NAMED_UNIT(*)
SI_UNIT(.CENTI.,.METRE.)
) ;
#50443=(
NAMED_UNIT(*)
PLANE_ANGLE_UNIT()
SI_UNIT($,.RADIAN.)
) ;
#50444=(
NAMED_UNIT(*)
SI_UNIT($,.STERADIAN.)
SOLID_ANGLE_UNIT()
) ;
#50470=SHAPE_DEFINITION_REPRESENTATION(#50546,#50644) ;
#50546=PRODUCT_DEFINITION_SHAPE('',$,#50697) ;
#50644=SHAPE_REPRESENTATION('',(#30734),#50413) ;
#50671=PRODUCT_DEFINITION_CONTEXT('part definition',#50829,'design') ;
#50697=PRODUCT_DEFINITION('METERING_GATE_ORIFICE_PLATE',
'METERING_GATE_ORIFICE_PLATE',#50749,#50671) ;
#50749=PRODUCT_DEFINITION_FORMATION('',$,#50856) ;
#50829=APPLICATION_CONTEXT(
'Core Data for Automotive Mechanical Design Process') ;
#50830=PRODUCT_CONTEXT('part definition',#50829,'mechanical') ;
#50856=PRODUCT('METERING_GATE_ORIFICE_PLATE','METERING_GATE_ORIFICE_PLATE',
$,(#50830)) ;
#50889=PRESENTATION_STYLE_ASSIGNMENT((#50896)) ;
#50896=SURFACE_STYLE_USAGE(.BOTH.,#50903) ;
#50903=SURFACE_SIDE_STYLE('',(#50910)) ;
#50910=SURFACE_STYLE_FILL_AREA(#50917) ;
#50917=FILL_AREA_STYLE('Stainless Steel - Satin',(#50924)) ;
#50924=FILL_AREA_STYLE_COLOUR('Stainless Steel - Satin',#50931) ;
#50931=COLOUR_RGB('Stainless Steel - Satin', 0.72549020, 0.75294118, 0.79215686) ;
ENDSEC;
END-ISO-10303-21;
